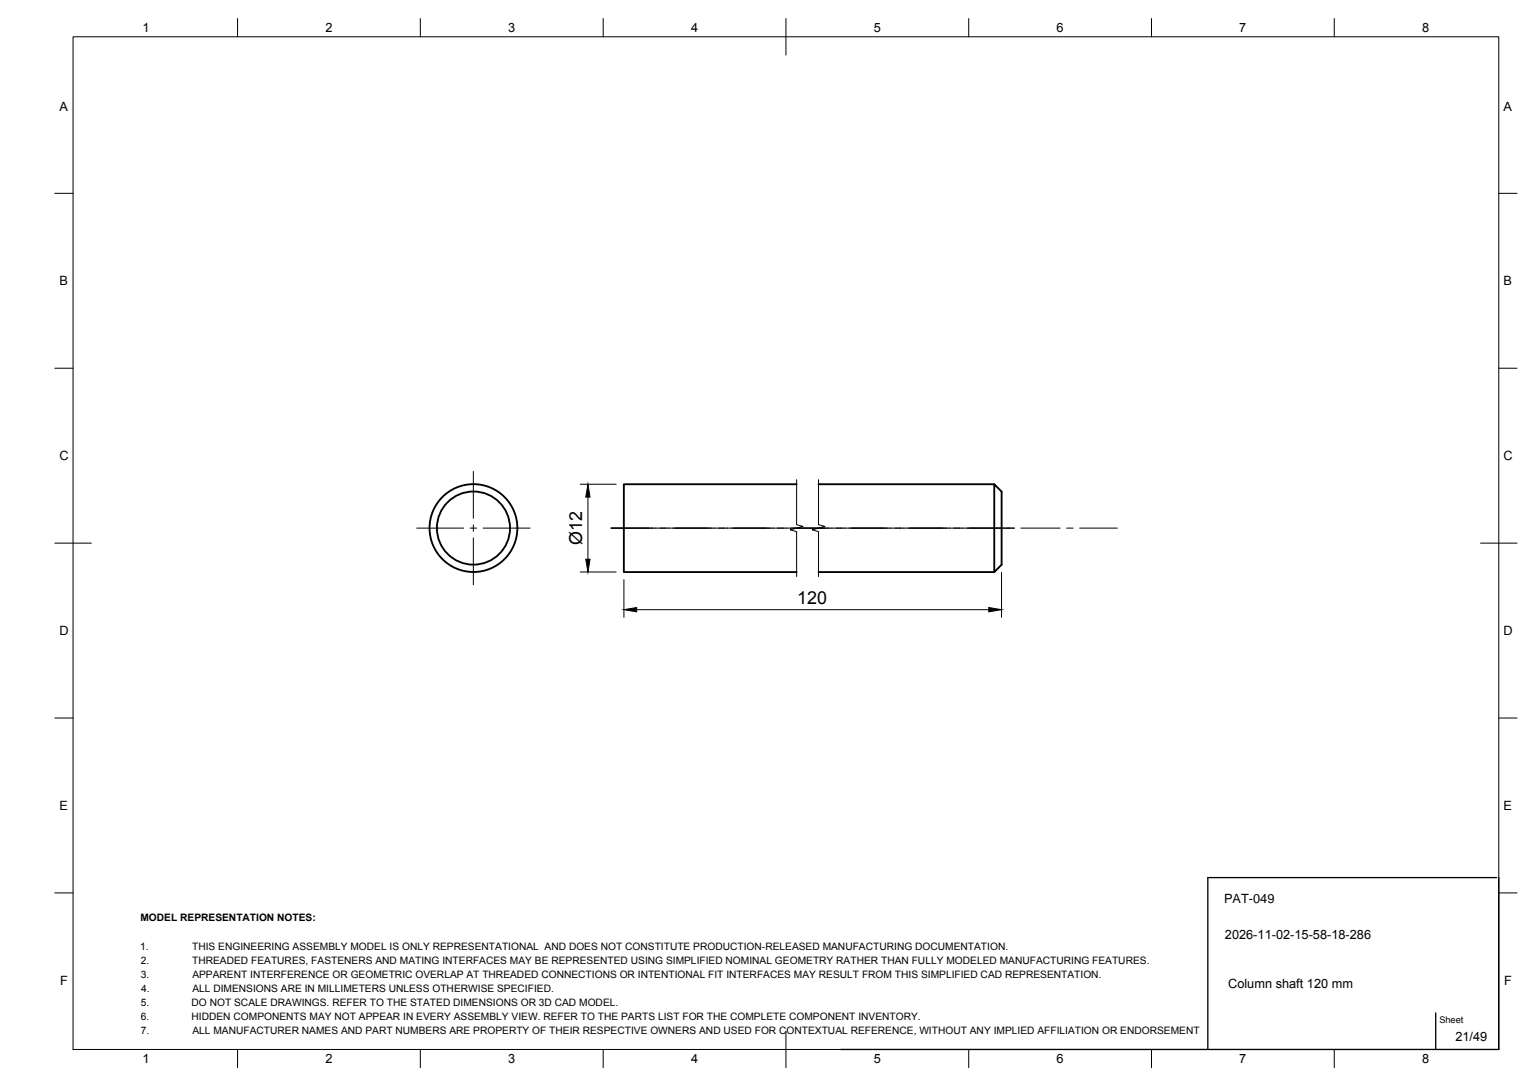
ISO-10303-21;
HEADER;
/* Generated by software containing ST-Developer
 * from STEP Tools, Inc. (www.steptools.com) 
 */

FILE_DESCRIPTION(
/* description */ ('Hand drill press frame (manual)'),
/* implementation_level */ '2;1');

FILE_NAME(
/* name */ 'Column shaft 120 mm.step',
/* time_stamp */ '2026-10-28T03:25:28-07:00',
/* author */ (''),
/* organization */ (''),
/* preprocessor_version */ 'ST-DEVELOPER v20.2',
/* originating_system */ 'Autodesk Translation Framework v15.17.0.0',
/* authorisation */ '');

FILE_SCHEMA (('AUTOMOTIVE_DESIGN { 1 0 10303 214 3 1 1 }'));
ENDSEC;

DATA;
#10=MECHANICAL_DESIGN_GEOMETRIC_PRESENTATION_REPRESENTATION('',(#635),#33299);
#473=CONICAL_SURFACE('',#13598,0.55,0.785398163397448);
#545=SHAPE_REPRESENTATION_RELATIONSHIP('SRR','None',#33504,#590);
#590=ADVANCED_BREP_SHAPE_REPRESENTATION('',(#687),#33266);
#635=STYLED_ITEM('',(#33814),#687);
#687=MANIFOLD_SOLID_BREP('Body1',#12653);
#1015=PLANE('',#13596);
#1016=PLANE('',#13602);
#1552=FACE_OUTER_BOUND('',#2357,.T.);
#1553=FACE_OUTER_BOUND('',#2358,.T.);
#1554=FACE_OUTER_BOUND('',#2359,.T.);
#1555=FACE_OUTER_BOUND('',#2360,.T.);
#2357=EDGE_LOOP('',(#9437));
#2358=EDGE_LOOP('',(#9438,#9439,#9440,#9441));
#2359=EDGE_LOOP('',(#9442,#9443,#9444,#9445));
#2360=EDGE_LOOP('',(#9446));
#3201=LINE('',#19159,#4366);
#3202=LINE('',#19162,#4367);
#4366=VECTOR('',#15508,0.55);
#4367=VECTOR('',#15513,0.6);
#5390=CIRCLE('',#13597,0.6);
#5391=CIRCLE('',#13599,0.6);
#5392=CIRCLE('',#13600,0.5);
#5952=VERTEX_POINT('',#19153);
#5953=VERTEX_POINT('',#19156);
#5954=VERTEX_POINT('',#19158);
#7247=EDGE_CURVE('',#5952,#5952,#5390,.T.);
#7248=EDGE_CURVE('',#5953,#5953,#5391,.T.);
#7249=EDGE_CURVE('',#5953,#5954,#3201,.T.);
#7250=EDGE_CURVE('',#5954,#5954,#5392,.T.);
#7251=EDGE_CURVE('',#5952,#5953,#3202,.T.);
#9437=ORIENTED_EDGE('',*,*,#7247,.F.);
#9438=ORIENTED_EDGE('',*,*,#7248,.T.);
#9439=ORIENTED_EDGE('',*,*,#7249,.T.);
#9440=ORIENTED_EDGE('',*,*,#7250,.T.);
#9441=ORIENTED_EDGE('',*,*,#7249,.F.);
#9442=ORIENTED_EDGE('',*,*,#7247,.T.);
#9443=ORIENTED_EDGE('',*,*,#7251,.T.);
#9444=ORIENTED_EDGE('',*,*,#7248,.F.);
#9445=ORIENTED_EDGE('',*,*,#7251,.F.);
#9446=ORIENTED_EDGE('',*,*,#7250,.F.);
#11870=CYLINDRICAL_SURFACE('',#13601,0.6);
#12161=ADVANCED_FACE('',(#1552),#1015,.T.);
#12162=ADVANCED_FACE('',(#1553),#473,.T.);
#12163=ADVANCED_FACE('',(#1554),#11870,.T.);
#12164=ADVANCED_FACE('',(#1555),#1016,.F.);
#12653=CLOSED_SHELL('',(#12161,#12162,#12163,#12164));
#13595=AXIS2_PLACEMENT_3D('',#19151,#15498,#15499);
#13596=AXIS2_PLACEMENT_3D('',#19152,#15500,#15501);
#13597=AXIS2_PLACEMENT_3D('',#19154,#15502,#15503);
#13598=AXIS2_PLACEMENT_3D('',#19155,#15504,#15505);
#13599=AXIS2_PLACEMENT_3D('',#19157,#15506,#15507);
#13600=AXIS2_PLACEMENT_3D('',#19160,#15509,#15510);
#13601=AXIS2_PLACEMENT_3D('',#19161,#15511,#15512);
#13602=AXIS2_PLACEMENT_3D('',#19163,#15514,#15515);
#15498=DIRECTION('axis',(0.,0.,1.));
#15499=DIRECTION('refdir',(1.,0.,0.));
#15500=DIRECTION('center_axis',(1.,0.,0.));
#15501=DIRECTION('ref_axis',(0.,0.,-1.));
#15502=DIRECTION('center_axis',(-1.,0.,0.));
#15503=DIRECTION('ref_axis',(0.,0.,-1.));
#15504=DIRECTION('center_axis',(1.,0.,0.));
#15505=DIRECTION('ref_axis',(0.,0.,-1.));
#15506=DIRECTION('center_axis',(-1.,0.,0.));
#15507=DIRECTION('ref_axis',(0.,0.,-1.));
#15508=DIRECTION('',(-0.707106781186548,8.65956056235493E-17,-0.707106781186547));
#15509=DIRECTION('center_axis',(1.,0.,0.));
#15510=DIRECTION('ref_axis',(0.,0.,-1.));
#15511=DIRECTION('center_axis',(1.,0.,0.));
#15512=DIRECTION('ref_axis',(0.,0.,-1.));
#15513=DIRECTION('',(-1.,0.,0.));
#15514=DIRECTION('center_axis',(1.,0.,0.));
#15515=DIRECTION('ref_axis',(0.,0.,-1.));
#19151=CARTESIAN_POINT('',(0.,0.,0.));
#19152=CARTESIAN_POINT('Origin',(12.,0.,0.));
#19153=CARTESIAN_POINT('',(12.,7.34788079488412E-17,0.6));
#19154=CARTESIAN_POINT('Origin',(12.,0.,0.));
#19155=CARTESIAN_POINT('Origin',(0.05,0.,0.));
#19156=CARTESIAN_POINT('',(0.1,7.34788079488412E-17,0.6));
#19157=CARTESIAN_POINT('Origin',(0.1,0.,0.));
#19158=CARTESIAN_POINT('',(0.,-6.12323399573677E-17,0.5));
#19159=CARTESIAN_POINT('',(0.05,-6.73555739531044E-17,0.55));
#19160=CARTESIAN_POINT('Origin',(0.,0.,0.));
#19161=CARTESIAN_POINT('Origin',(0.,0.,0.));
#19162=CARTESIAN_POINT('',(0.,-7.34788079488412E-17,0.6));
#19163=CARTESIAN_POINT('Origin',(0.,0.,0.));
#33214=UNCERTAINTY_MEASURE_WITH_UNIT(LENGTH_MEASURE(0.001),#33300,
'DISTANCE_ACCURACY_VALUE',
'Maximum model space distance between geometric entities at asserted c
onnectivities');
#33247=UNCERTAINTY_MEASURE_WITH_UNIT(LENGTH_MEASURE(0.001),#33300,
'DISTANCE_ACCURACY_VALUE',
'Maximum model space distance between geometric entities at asserted c
onnectivities');
#33266=(
GEOMETRIC_REPRESENTATION_CONTEXT(3)
GLOBAL_UNCERTAINTY_ASSIGNED_CONTEXT((#33214))
GLOBAL_UNIT_ASSIGNED_CONTEXT((#33300,#33302,#33303))
REPRESENTATION_CONTEXT('','3D')
);
#33299=(
GEOMETRIC_REPRESENTATION_CONTEXT(3)
GLOBAL_UNCERTAINTY_ASSIGNED_CONTEXT((#33247))
GLOBAL_UNIT_ASSIGNED_CONTEXT((#33300,#33302,#33303))
REPRESENTATION_CONTEXT('','3D')
);
#33300=(
LENGTH_UNIT()
NAMED_UNIT(*)
SI_UNIT(.CENTI.,.METRE.)
);
#33302=(
NAMED_UNIT(*)
PLANE_ANGLE_UNIT()
SI_UNIT($,.RADIAN.)
);
#33303=(
NAMED_UNIT(*)
SI_UNIT($,.STERADIAN.)
SOLID_ANGLE_UNIT()
);
#33322=SHAPE_DEFINITION_REPRESENTATION(#33373,#33504);
#33373=PRODUCT_DEFINITION_SHAPE('',$,#33556);
#33504=SHAPE_REPRESENTATION('',(#13595),#33266);
#33537=PRODUCT_DEFINITION_CONTEXT('part definition',#33692,'design');
#33556=PRODUCT_DEFINITION('Column shaft 120 mm','Column shaft 120 mm',#33607,
#33537);
#33607=PRODUCT_DEFINITION_FORMATION('',$,#33712);
#33692=APPLICATION_CONTEXT(
'Core Data for Automotive Mechanical Design Process');
#33693=PRODUCT_CONTEXT('part definition',#33692,'mechanical');
#33712=PRODUCT('Column shaft 120 mm','Column shaft 120 mm',
'Column shaft 120 mm',(#33693));
#33808=COLOUR_RGB('Grey',0.48,0.52,0.57);
#33809=FILL_AREA_STYLE_COLOUR('',#33808);
#33810=FILL_AREA_STYLE('',(#33809));
#33811=SURFACE_STYLE_FILL_AREA(#33810);
#33812=SURFACE_SIDE_STYLE('',(#33811));
#33813=SURFACE_STYLE_USAGE(.BOTH.,#33812);
#33814=PRESENTATION_STYLE_ASSIGNMENT((#33813));
ENDSEC;
END-ISO-10303-21;
